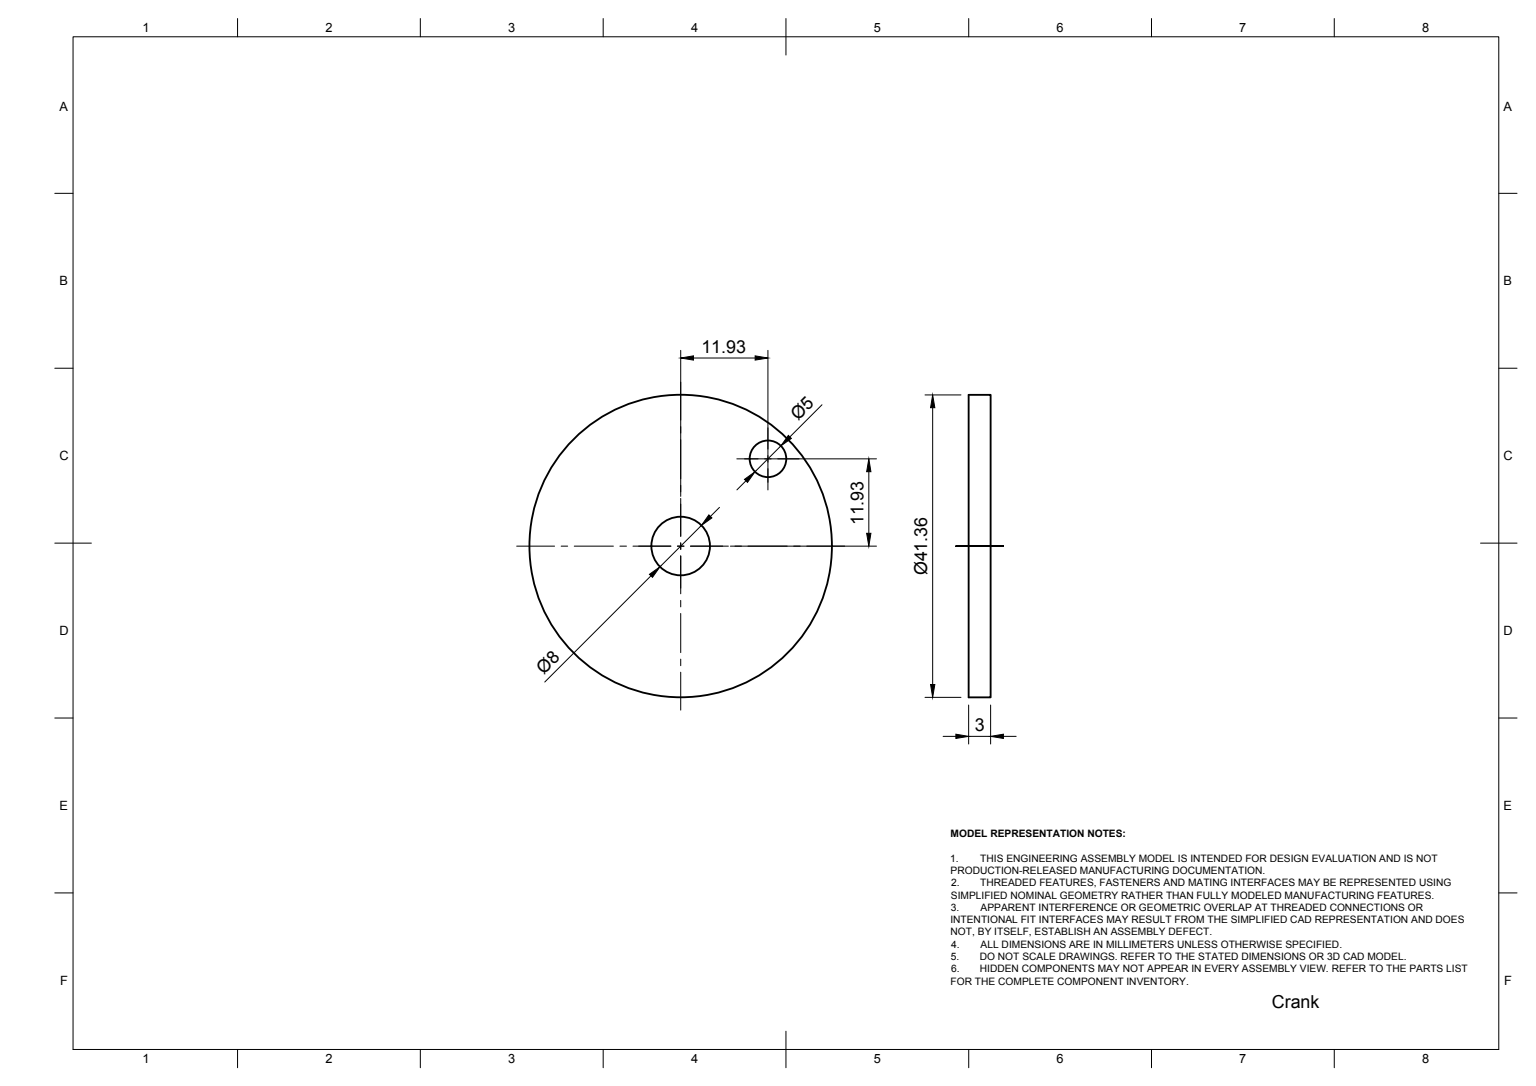
ISO-10303-21;
HEADER;
/* Generated by software containing ST-Developer
 * from STEP Tools, Inc. (www.steptools.com) 
 */

FILE_DESCRIPTION(
/* description */ (''),
/* implementation_level */ '2;1');

FILE_NAME(
/* name */ 'Crank.step',
/* time_stamp */ '2026-10-04T12:17:52-07:00',
/* author */ (''),
/* organization */ (''),
/* preprocessor_version */ 'ST-DEVELOPER v20.2',
/* originating_system */ 'Autodesk Translation Framework v15.15.0.0',
/* authorisation */ '');

FILE_SCHEMA (('AUTOMOTIVE_DESIGN { 1 0 10303 214 3 1 1 }'));
ENDSEC;

DATA;
#10=MECHANICAL_DESIGN_GEOMETRIC_PRESENTATION_REPRESENTATION('',(#68),#1602);
#52=SHAPE_REPRESENTATION_RELATIONSHIP('SRR','None',#1639,#60);
#60=ADVANCED_BREP_SHAPE_REPRESENTATION('',(#76),#1599);
#68=STYLED_ITEM('',(#1685),#76);
#76=MANIFOLD_SOLID_BREP('Body1',#779);
#87=FACE_BOUND('',#249,.T.);
#88=FACE_BOUND('',#250,.T.);
#89=FACE_BOUND('',#252,.T.);
#90=FACE_BOUND('',#253,.T.);
#121=CIRCLE('',#942,4.);
#122=CIRCLE('',#943,4.);
#123=CIRCLE('',#945,2.5);
#124=CIRCLE('',#946,2.5);
#125=CIRCLE('',#948,20.6801665756397);
#126=CIRCLE('',#949,20.6801665756397);
#149=CYLINDRICAL_SURFACE('',#941,4.);
#150=CYLINDRICAL_SURFACE('',#944,2.5);
#151=CYLINDRICAL_SURFACE('',#947,20.6801665756397);
#190=FACE_OUTER_BOUND('',#245,.T.);
#191=FACE_OUTER_BOUND('',#246,.T.);
#192=FACE_OUTER_BOUND('',#247,.T.);
#193=FACE_OUTER_BOUND('',#248,.T.);
#194=FACE_OUTER_BOUND('',#251,.T.);
#245=EDGE_LOOP('',(#666,#667,#668,#669));
#246=EDGE_LOOP('',(#670,#671,#672,#673));
#247=EDGE_LOOP('',(#674,#675,#676,#677));
#248=EDGE_LOOP('',(#678));
#249=EDGE_LOOP('',(#679));
#250=EDGE_LOOP('',(#680));
#251=EDGE_LOOP('',(#681));
#252=EDGE_LOOP('',(#682));
#253=EDGE_LOOP('',(#683));
#306=LINE('',#1535,#355);
#307=LINE('',#1541,#356);
#308=LINE('',#1547,#357);
#355=VECTOR('',#1162,4.);
#356=VECTOR('',#1169,2.5);
#357=VECTOR('',#1176,20.6801665756397);
#411=VERTEX_POINT('',#1532);
#412=VERTEX_POINT('',#1534);
#413=VERTEX_POINT('',#1538);
#414=VERTEX_POINT('',#1540);
#415=VERTEX_POINT('',#1544);
#416=VERTEX_POINT('',#1546);
#498=EDGE_CURVE('',#411,#411,#121,.T.);
#499=EDGE_CURVE('',#411,#412,#306,.T.);
#500=EDGE_CURVE('',#412,#412,#122,.T.);
#501=EDGE_CURVE('',#413,#413,#123,.T.);
#502=EDGE_CURVE('',#413,#414,#307,.T.);
#503=EDGE_CURVE('',#414,#414,#124,.T.);
#504=EDGE_CURVE('',#415,#415,#125,.T.);
#505=EDGE_CURVE('',#415,#416,#308,.T.);
#506=EDGE_CURVE('',#416,#416,#126,.T.);
#666=ORIENTED_EDGE('',*,*,#498,.F.);
#667=ORIENTED_EDGE('',*,*,#499,.T.);
#668=ORIENTED_EDGE('',*,*,#500,.F.);
#669=ORIENTED_EDGE('',*,*,#499,.F.);
#670=ORIENTED_EDGE('',*,*,#501,.F.);
#671=ORIENTED_EDGE('',*,*,#502,.T.);
#672=ORIENTED_EDGE('',*,*,#503,.F.);
#673=ORIENTED_EDGE('',*,*,#502,.F.);
#674=ORIENTED_EDGE('',*,*,#504,.F.);
#675=ORIENTED_EDGE('',*,*,#505,.T.);
#676=ORIENTED_EDGE('',*,*,#506,.T.);
#677=ORIENTED_EDGE('',*,*,#505,.F.);
#678=ORIENTED_EDGE('',*,*,#504,.T.);
#679=ORIENTED_EDGE('',*,*,#500,.T.);
#680=ORIENTED_EDGE('',*,*,#501,.T.);
#681=ORIENTED_EDGE('',*,*,#506,.F.);
#682=ORIENTED_EDGE('',*,*,#498,.T.);
#683=ORIENTED_EDGE('',*,*,#503,.T.);
#721=PLANE('',#950);
#722=PLANE('',#951);
#762=ADVANCED_FACE('',(#190),#149,.F.);
#763=ADVANCED_FACE('',(#191),#150,.F.);
#764=ADVANCED_FACE('',(#192),#151,.T.);
#765=ADVANCED_FACE('',(#193,#87,#88),#721,.T.);
#766=ADVANCED_FACE('',(#194,#89,#90),#722,.F.);
#779=CLOSED_SHELL('',(#762,#763,#764,#765,#766));
#940=AXIS2_PLACEMENT_3D('',#1530,#1156,#1157);
#941=AXIS2_PLACEMENT_3D('',#1531,#1158,#1159);
#942=AXIS2_PLACEMENT_3D('',#1533,#1160,#1161);
#943=AXIS2_PLACEMENT_3D('',#1536,#1163,#1164);
#944=AXIS2_PLACEMENT_3D('',#1537,#1165,#1166);
#945=AXIS2_PLACEMENT_3D('',#1539,#1167,#1168);
#946=AXIS2_PLACEMENT_3D('',#1542,#1170,#1171);
#947=AXIS2_PLACEMENT_3D('',#1543,#1172,#1173);
#948=AXIS2_PLACEMENT_3D('',#1545,#1174,#1175);
#949=AXIS2_PLACEMENT_3D('',#1548,#1177,#1178);
#950=AXIS2_PLACEMENT_3D('',#1549,#1179,#1180);
#951=AXIS2_PLACEMENT_3D('',#1550,#1181,#1182);
#1156=DIRECTION('axis',(0.,0.,1.));
#1157=DIRECTION('refdir',(1.,0.,0.));
#1158=DIRECTION('center_axis',(0.,1.,0.));
#1159=DIRECTION('ref_axis',(-1.,0.,0.));
#1160=DIRECTION('center_axis',(0.,1.,0.));
#1161=DIRECTION('ref_axis',(-1.,0.,0.));
#1162=DIRECTION('',(0.,1.,0.));
#1163=DIRECTION('center_axis',(0.,-1.,0.));
#1164=DIRECTION('ref_axis',(-1.,0.,0.));
#1165=DIRECTION('center_axis',(0.,-1.,0.));
#1166=DIRECTION('ref_axis',(1.,0.,0.));
#1167=DIRECTION('center_axis',(0.,-1.,0.));
#1168=DIRECTION('ref_axis',(1.,0.,0.));
#1169=DIRECTION('',(0.,-1.,0.));
#1170=DIRECTION('center_axis',(0.,1.,0.));
#1171=DIRECTION('ref_axis',(1.,0.,0.));
#1172=DIRECTION('center_axis',(0.,1.,0.));
#1173=DIRECTION('ref_axis',(1.,0.,0.));
#1174=DIRECTION('center_axis',(0.,1.,0.));
#1175=DIRECTION('ref_axis',(1.,0.,0.));
#1176=DIRECTION('',(0.,-1.,0.));
#1177=DIRECTION('center_axis',(0.,1.,0.));
#1178=DIRECTION('ref_axis',(1.,0.,0.));
#1179=DIRECTION('center_axis',(0.,1.,0.));
#1180=DIRECTION('ref_axis',(1.,0.,0.));
#1181=DIRECTION('center_axis',(0.,1.,0.));
#1182=DIRECTION('ref_axis',(1.,0.,0.));
#1530=CARTESIAN_POINT('',(0.,0.,0.));
#1531=CARTESIAN_POINT('Origin',(23.8627874897787,0.,50.));
#1532=CARTESIAN_POINT('',(27.8627874897787,-3.,50.));
#1533=CARTESIAN_POINT('Origin',(23.8627874897787,-3.,50.));
#1534=CARTESIAN_POINT('',(27.8627874897787,0.,50.));
#1535=CARTESIAN_POINT('',(27.8627874897787,0.,50.));
#1536=CARTESIAN_POINT('Origin',(23.8627874897787,0.,50.));
#1537=CARTESIAN_POINT('Origin',(11.9313937448893,-3.,61.9313937448893));
#1538=CARTESIAN_POINT('',(9.43139374488932,0.,61.9313937448893));
#1539=CARTESIAN_POINT('Origin',(11.9313937448893,0.,61.9313937448893));
#1540=CARTESIAN_POINT('',(9.43139374488932,-3.,61.9313937448893));
#1541=CARTESIAN_POINT('',(9.4313937448893,-3.,61.9313937448893));
#1542=CARTESIAN_POINT('Origin',(11.9313937448893,-3.,61.9313937448893));
#1543=CARTESIAN_POINT('Origin',(23.8627874897787,-3.,50.));
#1544=CARTESIAN_POINT('',(3.18262091413893,0.,50.));
#1545=CARTESIAN_POINT('Origin',(23.8627874897787,0.,50.));
#1546=CARTESIAN_POINT('',(3.18262091413893,-3.,50.));
#1547=CARTESIAN_POINT('',(3.182620914139,-3.,50.));
#1548=CARTESIAN_POINT('Origin',(23.8627874897787,-3.,50.));
#1549=CARTESIAN_POINT('Origin',(23.8627874897787,0.,50.));
#1550=CARTESIAN_POINT('Origin',(23.8627874897787,-3.,50.));
#1589=UNCERTAINTY_MEASURE_WITH_UNIT(LENGTH_MEASURE(0.01),#1603,
'DISTANCE_ACCURACY_VALUE',
'Maximum model space distance between geometric entities at asserted c
onnectivities');
#1592=UNCERTAINTY_MEASURE_WITH_UNIT(LENGTH_MEASURE(0.01),#1603,
'DISTANCE_ACCURACY_VALUE',
'Maximum model space distance between geometric entities at asserted c
onnectivities');
#1599=(
GEOMETRIC_REPRESENTATION_CONTEXT(3)
GLOBAL_UNCERTAINTY_ASSIGNED_CONTEXT((#1589))
GLOBAL_UNIT_ASSIGNED_CONTEXT((#1603,#1605,#1606))
REPRESENTATION_CONTEXT('','3D')
);
#1602=(
GEOMETRIC_REPRESENTATION_CONTEXT(3)
GLOBAL_UNCERTAINTY_ASSIGNED_CONTEXT((#1592))
GLOBAL_UNIT_ASSIGNED_CONTEXT((#1603,#1605,#1606))
REPRESENTATION_CONTEXT('','3D')
);
#1603=(
LENGTH_UNIT()
NAMED_UNIT(*)
SI_UNIT(.MILLI.,.METRE.)
);
#1605=(
NAMED_UNIT(*)
PLANE_ANGLE_UNIT()
SI_UNIT($,.RADIAN.)
);
#1606=(
NAMED_UNIT(*)
SI_UNIT($,.STERADIAN.)
SOLID_ANGLE_UNIT()
);
#1613=SHAPE_DEFINITION_REPRESENTATION(#1622,#1639);
#1622=PRODUCT_DEFINITION_SHAPE('',$,#1649);
#1639=SHAPE_REPRESENTATION('',(#940),#1599);
#1642=PRODUCT_DEFINITION_CONTEXT('part definition',#1671,'design');
#1649=PRODUCT_DEFINITION('Crank','Crank',#1658,#1642);
#1658=PRODUCT_DEFINITION_FORMATION('',$,#1679);
#1671=APPLICATION_CONTEXT(
'Core Data for Automotive Mechanical Design Process');
#1672=PRODUCT_CONTEXT('part definition',#1671,'mechanical');
#1679=PRODUCT('Crank','Crank',$,(#1672));
#1685=PRESENTATION_STYLE_ASSIGNMENT((#1689));
#1689=SURFACE_STYLE_USAGE(.BOTH.,#1693);
#1693=SURFACE_SIDE_STYLE('',(#1697));
#1697=SURFACE_STYLE_FILL_AREA(#1701);
#1701=FILL_AREA_STYLE('Opaque(85,255,0)',(#1705));
#1705=FILL_AREA_STYLE_COLOUR('Opaque(85,255,0)',#1709);
#1709=COLOUR_RGB('Opaque(85,255,0)', 0.40784314, 0.44705882, 0.49803922);
ENDSEC;
END-ISO-10303-21;
